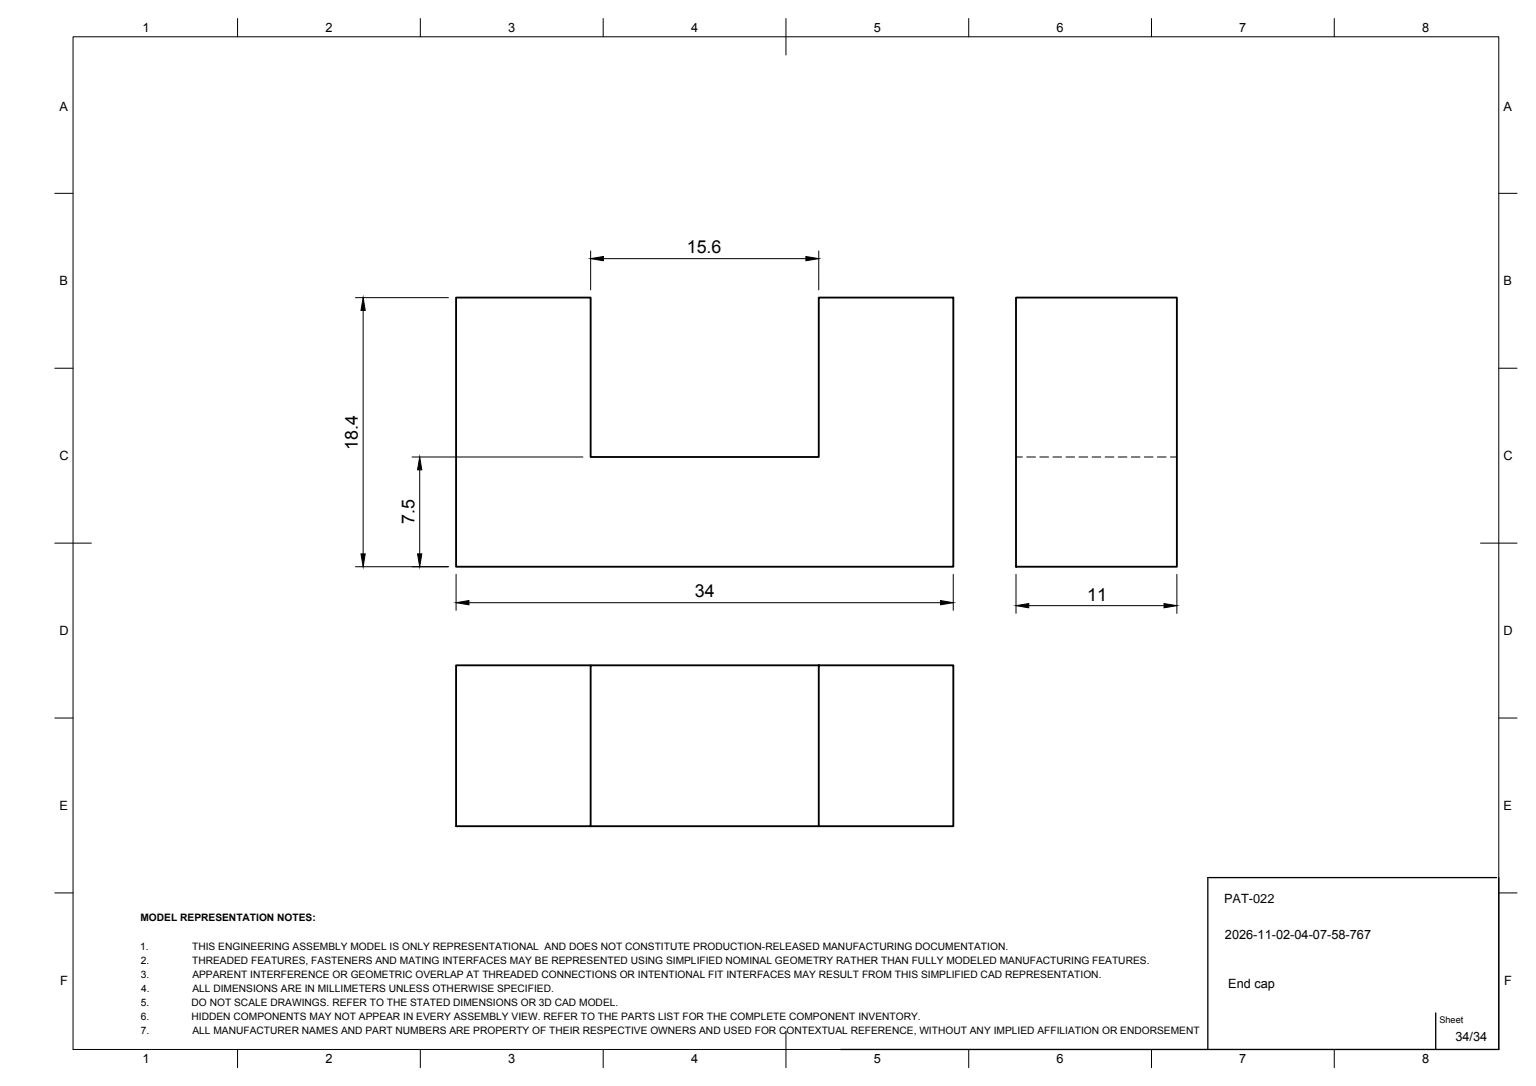
ISO-10303-21;
HEADER;
/* Generated by software containing ST-Developer
 * from STEP Tools, Inc. (www.steptools.com) 
 */

FILE_DESCRIPTION(
/* description */ ('Chute with adjustable gate'),
/* implementation_level */ '2;1');

FILE_NAME(
/* name */ 'End cap.step',
/* time_stamp */ '2026-10-27T10:52:28-07:00',
/* author */ (''),
/* organization */ (''),
/* preprocessor_version */ 'ST-DEVELOPER v20.2',
/* originating_system */ 'Autodesk Translation Framework v15.17.0.0',
/* authorisation */ '');

FILE_SCHEMA (('AUTOMOTIVE_DESIGN { 1 0 10303 214 3 1 1 }'));
ENDSEC;

DATA;
#10=MECHANICAL_DESIGN_GEOMETRIC_PRESENTATION_REPRESENTATION('',(#443),#13094);
#379=SHAPE_REPRESENTATION_RELATIONSHIP('SRR','None',#13282,#411);
#411=ADVANCED_BREP_SHAPE_REPRESENTATION('',(#473),#13091);
#443=STYLED_ITEM('',(#13509),#473);
#473=MANIFOLD_SOLID_BREP('Body1',#7628);
#882=PLANE('',#8560);
#883=PLANE('',#8561);
#884=PLANE('',#8562);
#885=PLANE('',#8563);
#886=PLANE('',#8564);
#887=PLANE('',#8565);
#888=PLANE('',#8566);
#889=PLANE('',#8567);
#890=PLANE('',#8568);
#891=PLANE('',#8569);
#1286=FACE_OUTER_BOUND('',#1815,.T.);
#1287=FACE_OUTER_BOUND('',#1816,.T.);
#1288=FACE_OUTER_BOUND('',#1817,.T.);
#1289=FACE_OUTER_BOUND('',#1818,.T.);
#1290=FACE_OUTER_BOUND('',#1819,.T.);
#1291=FACE_OUTER_BOUND('',#1820,.T.);
#1292=FACE_OUTER_BOUND('',#1821,.T.);
#1293=FACE_OUTER_BOUND('',#1822,.T.);
#1294=FACE_OUTER_BOUND('',#1823,.T.);
#1295=FACE_OUTER_BOUND('',#1824,.T.);
#1815=EDGE_LOOP('',(#6934,#6935,#6936,#6937));
#1816=EDGE_LOOP('',(#6938,#6939,#6940,#6941));
#1817=EDGE_LOOP('',(#6942,#6943,#6944,#6945));
#1818=EDGE_LOOP('',(#6946,#6947,#6948,#6949));
#1819=EDGE_LOOP('',(#6950,#6951,#6952,#6953));
#1820=EDGE_LOOP('',(#6954,#6955,#6956,#6957));
#1821=EDGE_LOOP('',(#6958,#6959,#6960,#6961));
#1822=EDGE_LOOP('',(#6962,#6963,#6964,#6965));
#1823=EDGE_LOOP('',(#6966,#6967,#6968,#6969,#6970,#6971,#6972,#6973));
#1824=EDGE_LOOP('',(#6974,#6975,#6976,#6977,#6978,#6979,#6980,#6981));
#2566=LINE('',#12760,#3343);
#2567=LINE('',#12762,#3344);
#2568=LINE('',#12764,#3345);
#2569=LINE('',#12765,#3346);
#2570=LINE('',#12768,#3347);
#2571=LINE('',#12770,#3348);
#2572=LINE('',#12771,#3349);
#2573=LINE('',#12774,#3350);
#2574=LINE('',#12776,#3351);
#2575=LINE('',#12777,#3352);
#2576=LINE('',#12780,#3353);
#2577=LINE('',#12782,#3354);
#2578=LINE('',#12783,#3355);
#2579=LINE('',#12786,#3356);
#2580=LINE('',#12788,#3357);
#2581=LINE('',#12789,#3358);
#2582=LINE('',#12792,#3359);
#2583=LINE('',#12794,#3360);
#2584=LINE('',#12795,#3361);
#2585=LINE('',#12798,#3362);
#2586=LINE('',#12800,#3363);
#2587=LINE('',#12801,#3364);
#2588=LINE('',#12803,#3365);
#2589=LINE('',#12804,#3366);
#3343=VECTOR('',#10554,1.);
#3344=VECTOR('',#10555,1.);
#3345=VECTOR('',#10556,1.);
#3346=VECTOR('',#10557,1.);
#3347=VECTOR('',#10560,1.);
#3348=VECTOR('',#10561,1.);
#3349=VECTOR('',#10562,1.);
#3350=VECTOR('',#10565,1.);
#3351=VECTOR('',#10566,1.);
#3352=VECTOR('',#10567,1.);
#3353=VECTOR('',#10570,1.);
#3354=VECTOR('',#10571,1.);
#3355=VECTOR('',#10572,1.);
#3356=VECTOR('',#10575,1.);
#3357=VECTOR('',#10576,1.);
#3358=VECTOR('',#10577,1.);
#3359=VECTOR('',#10580,1.);
#3360=VECTOR('',#10581,1.);
#3361=VECTOR('',#10582,1.);
#3362=VECTOR('',#10585,1.);
#3363=VECTOR('',#10586,1.);
#3364=VECTOR('',#10587,1.);
#3365=VECTOR('',#10590,1.);
#3366=VECTOR('',#10591,1.);
#4171=VERTEX_POINT('',#12758);
#4172=VERTEX_POINT('',#12759);
#4173=VERTEX_POINT('',#12761);
#4174=VERTEX_POINT('',#12763);
#4175=VERTEX_POINT('',#12767);
#4176=VERTEX_POINT('',#12769);
#4177=VERTEX_POINT('',#12773);
#4178=VERTEX_POINT('',#12775);
#4179=VERTEX_POINT('',#12779);
#4180=VERTEX_POINT('',#12781);
#4181=VERTEX_POINT('',#12785);
#4182=VERTEX_POINT('',#12787);
#4183=VERTEX_POINT('',#12791);
#4184=VERTEX_POINT('',#12793);
#4185=VERTEX_POINT('',#12797);
#4186=VERTEX_POINT('',#12799);
#5100=EDGE_CURVE('',#4171,#4172,#2566,.T.);
#5101=EDGE_CURVE('',#4171,#4173,#2567,.T.);
#5102=EDGE_CURVE('',#4174,#4173,#2568,.T.);
#5103=EDGE_CURVE('',#4172,#4174,#2569,.T.);
#5104=EDGE_CURVE('',#4172,#4175,#2570,.T.);
#5105=EDGE_CURVE('',#4176,#4174,#2571,.T.);
#5106=EDGE_CURVE('',#4175,#4176,#2572,.T.);
#5107=EDGE_CURVE('',#4175,#4177,#2573,.T.);
#5108=EDGE_CURVE('',#4178,#4176,#2574,.T.);
#5109=EDGE_CURVE('',#4177,#4178,#2575,.T.);
#5110=EDGE_CURVE('',#4177,#4179,#2576,.T.);
#5111=EDGE_CURVE('',#4180,#4178,#2577,.T.);
#5112=EDGE_CURVE('',#4179,#4180,#2578,.T.);
#5113=EDGE_CURVE('',#4179,#4181,#2579,.T.);
#5114=EDGE_CURVE('',#4182,#4180,#2580,.T.);
#5115=EDGE_CURVE('',#4181,#4182,#2581,.T.);
#5116=EDGE_CURVE('',#4181,#4183,#2582,.T.);
#5117=EDGE_CURVE('',#4184,#4182,#2583,.T.);
#5118=EDGE_CURVE('',#4183,#4184,#2584,.T.);
#5119=EDGE_CURVE('',#4183,#4185,#2585,.T.);
#5120=EDGE_CURVE('',#4186,#4184,#2586,.T.);
#5121=EDGE_CURVE('',#4185,#4186,#2587,.T.);
#5122=EDGE_CURVE('',#4185,#4171,#2588,.T.);
#5123=EDGE_CURVE('',#4173,#4186,#2589,.T.);
#6934=ORIENTED_EDGE('',*,*,#5100,.F.);
#6935=ORIENTED_EDGE('',*,*,#5101,.T.);
#6936=ORIENTED_EDGE('',*,*,#5102,.F.);
#6937=ORIENTED_EDGE('',*,*,#5103,.F.);
#6938=ORIENTED_EDGE('',*,*,#5104,.F.);
#6939=ORIENTED_EDGE('',*,*,#5103,.T.);
#6940=ORIENTED_EDGE('',*,*,#5105,.F.);
#6941=ORIENTED_EDGE('',*,*,#5106,.F.);
#6942=ORIENTED_EDGE('',*,*,#5107,.F.);
#6943=ORIENTED_EDGE('',*,*,#5106,.T.);
#6944=ORIENTED_EDGE('',*,*,#5108,.F.);
#6945=ORIENTED_EDGE('',*,*,#5109,.F.);
#6946=ORIENTED_EDGE('',*,*,#5110,.F.);
#6947=ORIENTED_EDGE('',*,*,#5109,.T.);
#6948=ORIENTED_EDGE('',*,*,#5111,.F.);
#6949=ORIENTED_EDGE('',*,*,#5112,.F.);
#6950=ORIENTED_EDGE('',*,*,#5113,.F.);
#6951=ORIENTED_EDGE('',*,*,#5112,.T.);
#6952=ORIENTED_EDGE('',*,*,#5114,.F.);
#6953=ORIENTED_EDGE('',*,*,#5115,.F.);
#6954=ORIENTED_EDGE('',*,*,#5116,.F.);
#6955=ORIENTED_EDGE('',*,*,#5115,.T.);
#6956=ORIENTED_EDGE('',*,*,#5117,.F.);
#6957=ORIENTED_EDGE('',*,*,#5118,.F.);
#6958=ORIENTED_EDGE('',*,*,#5119,.F.);
#6959=ORIENTED_EDGE('',*,*,#5118,.T.);
#6960=ORIENTED_EDGE('',*,*,#5120,.F.);
#6961=ORIENTED_EDGE('',*,*,#5121,.F.);
#6962=ORIENTED_EDGE('',*,*,#5122,.F.);
#6963=ORIENTED_EDGE('',*,*,#5121,.T.);
#6964=ORIENTED_EDGE('',*,*,#5123,.F.);
#6965=ORIENTED_EDGE('',*,*,#5101,.F.);
#6966=ORIENTED_EDGE('',*,*,#5122,.T.);
#6967=ORIENTED_EDGE('',*,*,#5100,.T.);
#6968=ORIENTED_EDGE('',*,*,#5104,.T.);
#6969=ORIENTED_EDGE('',*,*,#5107,.T.);
#6970=ORIENTED_EDGE('',*,*,#5110,.T.);
#6971=ORIENTED_EDGE('',*,*,#5113,.T.);
#6972=ORIENTED_EDGE('',*,*,#5116,.T.);
#6973=ORIENTED_EDGE('',*,*,#5119,.T.);
#6974=ORIENTED_EDGE('',*,*,#5123,.T.);
#6975=ORIENTED_EDGE('',*,*,#5120,.T.);
#6976=ORIENTED_EDGE('',*,*,#5117,.T.);
#6977=ORIENTED_EDGE('',*,*,#5114,.T.);
#6978=ORIENTED_EDGE('',*,*,#5111,.T.);
#6979=ORIENTED_EDGE('',*,*,#5108,.T.);
#6980=ORIENTED_EDGE('',*,*,#5105,.T.);
#6981=ORIENTED_EDGE('',*,*,#5102,.T.);
#7554=ADVANCED_FACE('',(#1286),#882,.T.);
#7555=ADVANCED_FACE('',(#1287),#883,.T.);
#7556=ADVANCED_FACE('',(#1288),#884,.T.);
#7557=ADVANCED_FACE('',(#1289),#885,.T.);
#7558=ADVANCED_FACE('',(#1290),#886,.T.);
#7559=ADVANCED_FACE('',(#1291),#887,.T.);
#7560=ADVANCED_FACE('',(#1292),#888,.T.);
#7561=ADVANCED_FACE('',(#1293),#889,.T.);
#7562=ADVANCED_FACE('',(#1294),#890,.T.);
#7563=ADVANCED_FACE('',(#1295),#891,.T.);
#7628=CLOSED_SHELL('',(#7554,#7555,#7556,#7557,#7558,#7559,#7560,#7561,
#7562,#7563));
#8559=AXIS2_PLACEMENT_3D('',#12756,#10550,#10551);
#8560=AXIS2_PLACEMENT_3D('',#12757,#10552,#10553);
#8561=AXIS2_PLACEMENT_3D('',#12766,#10558,#10559);
#8562=AXIS2_PLACEMENT_3D('',#12772,#10563,#10564);
#8563=AXIS2_PLACEMENT_3D('',#12778,#10568,#10569);
#8564=AXIS2_PLACEMENT_3D('',#12784,#10573,#10574);
#8565=AXIS2_PLACEMENT_3D('',#12790,#10578,#10579);
#8566=AXIS2_PLACEMENT_3D('',#12796,#10583,#10584);
#8567=AXIS2_PLACEMENT_3D('',#12802,#10588,#10589);
#8568=AXIS2_PLACEMENT_3D('',#12805,#10592,#10593);
#8569=AXIS2_PLACEMENT_3D('',#12806,#10594,#10595);
#10550=DIRECTION('axis',(0.,0.,1.));
#10551=DIRECTION('refdir',(1.,0.,0.));
#10552=DIRECTION('center_axis',(0.,0.,-1.));
#10553=DIRECTION('ref_axis',(0.,-1.,0.));
#10554=DIRECTION('',(0.,1.,0.));
#10555=DIRECTION('',(-1.,0.,0.));
#10556=DIRECTION('',(0.,-1.,0.));
#10557=DIRECTION('',(-1.,0.,0.));
#10558=DIRECTION('center_axis',(0.,1.,0.));
#10559=DIRECTION('ref_axis',(0.,0.,-1.));
#10560=DIRECTION('',(0.,0.,1.));
#10561=DIRECTION('',(0.,0.,-1.));
#10562=DIRECTION('',(-1.,0.,0.));
#10563=DIRECTION('center_axis',(0.,0.,-1.));
#10564=DIRECTION('ref_axis',(0.,-1.,0.));
#10565=DIRECTION('',(0.,1.,0.));
#10566=DIRECTION('',(0.,-1.,0.));
#10567=DIRECTION('',(-1.,0.,0.));
#10568=DIRECTION('center_axis',(0.,-1.,0.));
#10569=DIRECTION('ref_axis',(0.,0.,1.));
#10570=DIRECTION('',(0.,0.,-1.));
#10571=DIRECTION('',(0.,0.,1.));
#10572=DIRECTION('',(-1.,0.,0.));
#10573=DIRECTION('center_axis',(0.,0.,-1.));
#10574=DIRECTION('ref_axis',(0.,-1.,0.));
#10575=DIRECTION('',(0.,1.,0.));
#10576=DIRECTION('',(0.,-1.,0.));
#10577=DIRECTION('',(-1.,0.,0.));
#10578=DIRECTION('center_axis',(0.,1.,0.));
#10579=DIRECTION('ref_axis',(0.,0.,-1.));
#10580=DIRECTION('',(0.,0.,1.));
#10581=DIRECTION('',(0.,0.,-1.));
#10582=DIRECTION('',(-1.,0.,0.));
#10583=DIRECTION('center_axis',(0.,0.,1.));
#10584=DIRECTION('ref_axis',(0.,1.,0.));
#10585=DIRECTION('',(0.,-1.,0.));
#10586=DIRECTION('',(0.,1.,0.));
#10587=DIRECTION('',(-1.,0.,0.));
#10588=DIRECTION('center_axis',(0.,-1.,0.));
#10589=DIRECTION('ref_axis',(0.,0.,1.));
#10590=DIRECTION('',(0.,0.,-1.));
#10591=DIRECTION('',(0.,0.,1.));
#10592=DIRECTION('center_axis',(1.,0.,0.));
#10593=DIRECTION('ref_axis',(0.,0.,-1.));
#10594=DIRECTION('center_axis',(-1.,0.,0.));
#10595=DIRECTION('ref_axis',(0.,0.,1.));
#12756=CARTESIAN_POINT('',(0.,0.,0.));
#12757=CARTESIAN_POINT('Origin',(-1.97,-0.78,0.46));
#12758=CARTESIAN_POINT('',(-1.97,-1.7,0.46));
#12759=CARTESIAN_POINT('',(-1.97,-0.78,0.46));
#12760=CARTESIAN_POINT('',(-1.97,-1.7,0.46));
#12761=CARTESIAN_POINT('',(-3.07,-1.7,0.46));
#12762=CARTESIAN_POINT('',(-1.97,-1.7,0.46));
#12763=CARTESIAN_POINT('',(-3.07,-0.78,0.46));
#12764=CARTESIAN_POINT('',(-3.07,-1.7,0.46));
#12765=CARTESIAN_POINT('',(-1.97,-0.78,0.46));
#12766=CARTESIAN_POINT('Origin',(-1.97,-0.78,1.55));
#12767=CARTESIAN_POINT('',(-1.97,-0.78,1.55));
#12768=CARTESIAN_POINT('',(-1.97,-0.78,0.46));
#12769=CARTESIAN_POINT('',(-3.07,-0.78,1.55));
#12770=CARTESIAN_POINT('',(-3.07,-0.78,0.46));
#12771=CARTESIAN_POINT('',(-1.97,-0.78,1.55));
#12772=CARTESIAN_POINT('Origin',(-1.97,0.78,1.55));
#12773=CARTESIAN_POINT('',(-1.97,0.78,1.55));
#12774=CARTESIAN_POINT('',(-1.97,-0.78,1.55));
#12775=CARTESIAN_POINT('',(-3.07,0.78,1.55));
#12776=CARTESIAN_POINT('',(-3.07,-0.78,1.55));
#12777=CARTESIAN_POINT('',(-1.97,0.78,1.55));
#12778=CARTESIAN_POINT('Origin',(-1.97,0.78,0.46));
#12779=CARTESIAN_POINT('',(-1.97,0.78,0.46));
#12780=CARTESIAN_POINT('',(-1.97,0.78,1.55));
#12781=CARTESIAN_POINT('',(-3.07,0.78,0.46));
#12782=CARTESIAN_POINT('',(-3.07,0.78,1.55));
#12783=CARTESIAN_POINT('',(-1.97,0.78,0.46));
#12784=CARTESIAN_POINT('Origin',(-1.97,1.7,0.46));
#12785=CARTESIAN_POINT('',(-1.97,1.7,0.46));
#12786=CARTESIAN_POINT('',(-1.97,0.78,0.46));
#12787=CARTESIAN_POINT('',(-3.07,1.7,0.46));
#12788=CARTESIAN_POINT('',(-3.07,0.78,0.46));
#12789=CARTESIAN_POINT('',(-1.97,1.7,0.46));
#12790=CARTESIAN_POINT('Origin',(-1.97,1.7,2.3));
#12791=CARTESIAN_POINT('',(-1.97,1.7,2.3));
#12792=CARTESIAN_POINT('',(-1.97,1.7,0.46));
#12793=CARTESIAN_POINT('',(-3.07,1.7,2.3));
#12794=CARTESIAN_POINT('',(-3.07,1.7,0.46));
#12795=CARTESIAN_POINT('',(-1.97,1.7,2.3));
#12796=CARTESIAN_POINT('Origin',(-1.97,-1.7,2.3));
#12797=CARTESIAN_POINT('',(-1.97,-1.7,2.3));
#12798=CARTESIAN_POINT('',(-1.97,1.7,2.3));
#12799=CARTESIAN_POINT('',(-3.07,-1.7,2.3));
#12800=CARTESIAN_POINT('',(-3.07,1.7,2.3));
#12801=CARTESIAN_POINT('',(-1.97,-1.7,2.3));
#12802=CARTESIAN_POINT('Origin',(-1.97,-1.7,0.46));
#12803=CARTESIAN_POINT('',(-1.97,-1.7,2.3));
#12804=CARTESIAN_POINT('',(-3.07,-1.7,2.3));
#12805=CARTESIAN_POINT('Origin',(-1.97,0.,1.38));
#12806=CARTESIAN_POINT('Origin',(-3.07,0.,1.38));
#13054=UNCERTAINTY_MEASURE_WITH_UNIT(LENGTH_MEASURE(0.001),#13095,
'DISTANCE_ACCURACY_VALUE',
'Maximum model space distance between geometric entities at asserted c
onnectivities');
#13057=UNCERTAINTY_MEASURE_WITH_UNIT(LENGTH_MEASURE(0.001),#13095,
'DISTANCE_ACCURACY_VALUE',
'Maximum model space distance between geometric entities at asserted c
onnectivities');
#13091=(
GEOMETRIC_REPRESENTATION_CONTEXT(3)
GLOBAL_UNCERTAINTY_ASSIGNED_CONTEXT((#13054))
GLOBAL_UNIT_ASSIGNED_CONTEXT((#13095,#13097,#13098))
REPRESENTATION_CONTEXT('','3D')
);
#13094=(
GEOMETRIC_REPRESENTATION_CONTEXT(3)
GLOBAL_UNCERTAINTY_ASSIGNED_CONTEXT((#13057))
GLOBAL_UNIT_ASSIGNED_CONTEXT((#13095,#13097,#13098))
REPRESENTATION_CONTEXT('','3D')
);
#13095=(
LENGTH_UNIT()
NAMED_UNIT(*)
SI_UNIT(.CENTI.,.METRE.)
);
#13097=(
NAMED_UNIT(*)
PLANE_ANGLE_UNIT()
SI_UNIT($,.RADIAN.)
);
#13098=(
NAMED_UNIT(*)
SI_UNIT($,.STERADIAN.)
SOLID_ANGLE_UNIT()
);
#13132=SHAPE_DEFINITION_REPRESENTATION(#13168,#13282);
#13168=PRODUCT_DEFINITION_SHAPE('',$,#13319);
#13282=SHAPE_REPRESENTATION('',(#8559),#13091);
#13285=PRODUCT_DEFINITION_CONTEXT('part definition',#13395,'design');
#13319=PRODUCT_DEFINITION('End cap','End cap',#13355,#13285);
#13355=PRODUCT_DEFINITION_FORMATION('',$,#13430);
#13395=APPLICATION_CONTEXT(
'Core Data for Automotive Mechanical Design Process');
#13396=PRODUCT_CONTEXT('part definition',#13395,'mechanical');
#13430=PRODUCT('End cap','End cap','End cap',(#13396));
#13503=COLOUR_RGB('Off White',0.89,0.88,0.83);
#13504=FILL_AREA_STYLE_COLOUR('',#13503);
#13505=FILL_AREA_STYLE('',(#13504));
#13506=SURFACE_STYLE_FILL_AREA(#13505);
#13507=SURFACE_SIDE_STYLE('',(#13506));
#13508=SURFACE_STYLE_USAGE(.BOTH.,#13507);
#13509=PRESENTATION_STYLE_ASSIGNMENT((#13508));
ENDSEC;
END-ISO-10303-21;
